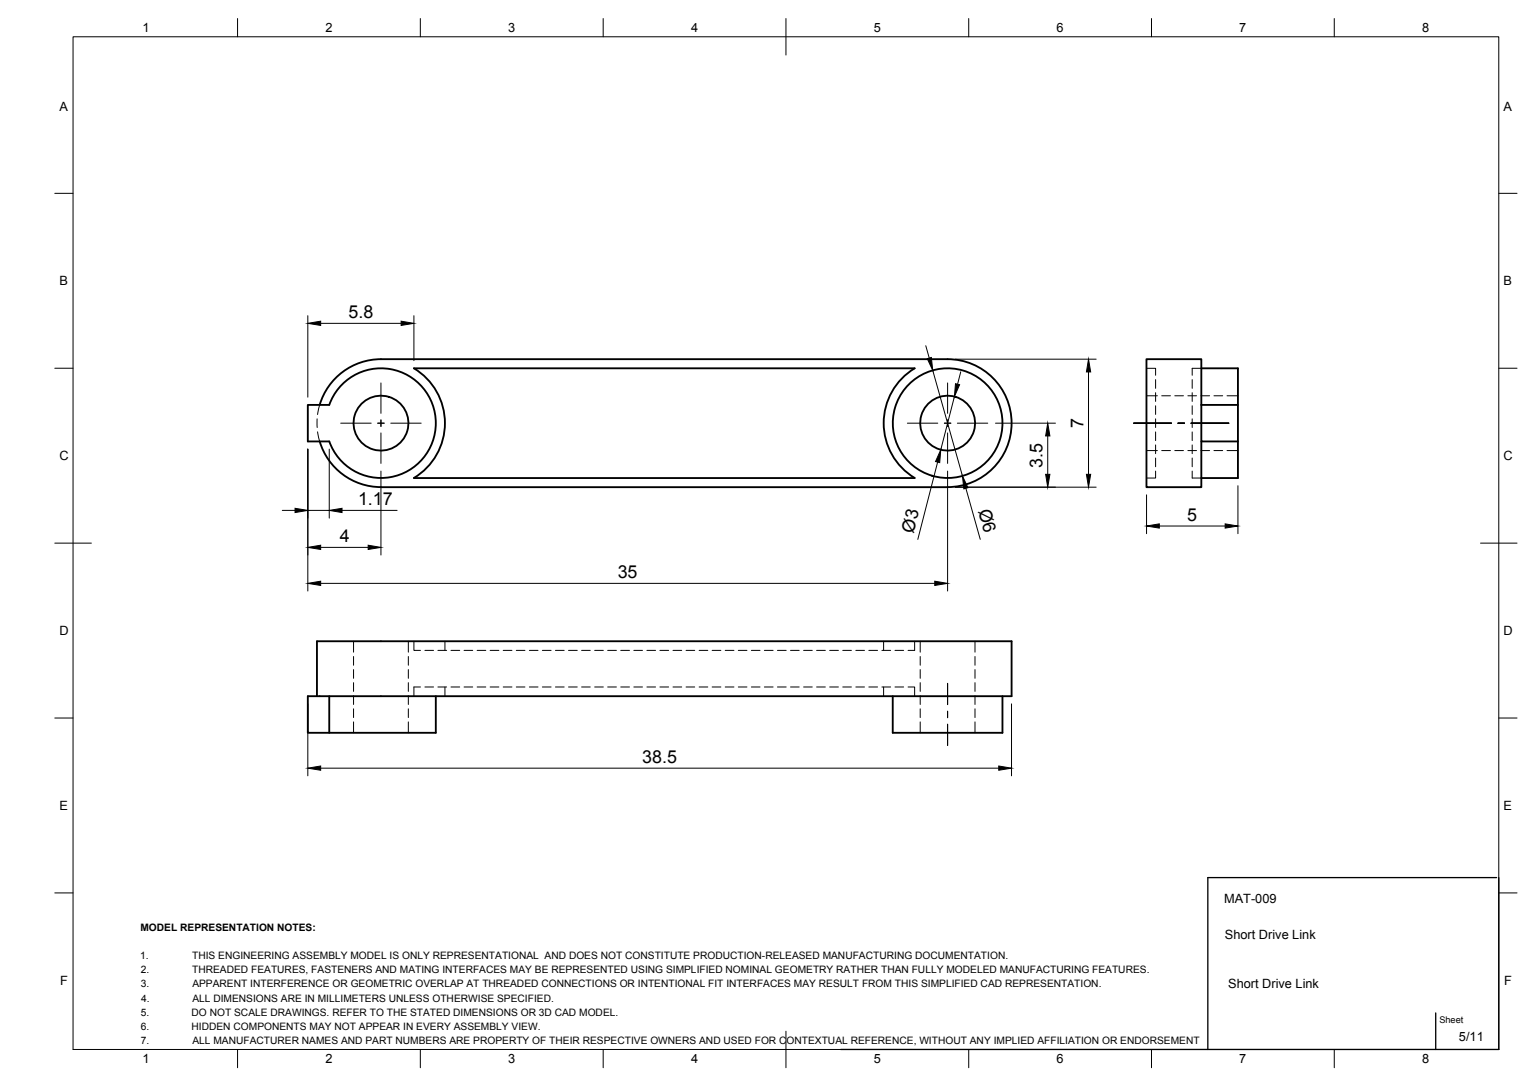
ISO-10303-21;
HEADER;
/* Generated by software containing ST-Developer
 * from STEP Tools, Inc. (www.steptools.com) 
 */

FILE_DESCRIPTION(
/* description */ ('STEP AP214'),
/* implementation_level */ '2;1');

FILE_NAME(
/* name */ 'Short Drive Link.step',
/* time_stamp */ '2026-11-14T05:43:09-08:00',
/* author */ (''),
/* organization */ (''),
/* preprocessor_version */ 'ST-DEVELOPER v20.2',
/* originating_system */ 'Autodesk Translation Framework v15.17.0.0',
/* authorisation */ '');

FILE_SCHEMA (('AUTOMOTIVE_DESIGN { 1 0 10303 214 3 1 1 }'));
ENDSEC;

DATA;
#10=MECHANICAL_DESIGN_GEOMETRIC_PRESENTATION_REPRESENTATION('',(#147),#11933);
#129=SHAPE_REPRESENTATION_RELATIONSHIP('SRR','None',#11989,#138);
#138=ADVANCED_BREP_SHAPE_REPRESENTATION('',(#156),#11925);
#147=STYLED_ITEM('',(#12042),#156);
#156=MANIFOLD_SOLID_BREP('Body1',#6644);
#176=FACE_BOUND('',#714,.T.);
#177=FACE_BOUND('',#715,.T.);
#178=FACE_BOUND('',#717,.T.);
#179=FACE_BOUND('',#718,.T.);
#180=FACE_BOUND('',#719,.T.);
#181=FACE_BOUND('',#737,.T.);
#182=FACE_BOUND('',#739,.T.);
#219=PLANE('',#6821);
#220=PLANE('',#6825);
#221=PLANE('',#6828);
#222=PLANE('',#6830);
#223=PLANE('',#6833);
#224=PLANE('',#6834);
#225=PLANE('',#6835);
#226=PLANE('',#6836);
#227=PLANE('',#6839);
#228=PLANE('',#6840);
#229=PLANE('',#6841);
#230=PLANE('',#6842);
#231=PLANE('',#6845);
#232=PLANE('',#6846);
#233=PLANE('',#6847);
#234=PLANE('',#6848);
#341=FACE_OUTER_BOUND('',#707,.T.);
#342=FACE_OUTER_BOUND('',#708,.T.);
#343=FACE_OUTER_BOUND('',#709,.T.);
#344=FACE_OUTER_BOUND('',#710,.T.);
#345=FACE_OUTER_BOUND('',#711,.T.);
#346=FACE_OUTER_BOUND('',#712,.T.);
#347=FACE_OUTER_BOUND('',#713,.T.);
#348=FACE_OUTER_BOUND('',#716,.T.);
#349=FACE_OUTER_BOUND('',#720,.T.);
#350=FACE_OUTER_BOUND('',#721,.T.);
#351=FACE_OUTER_BOUND('',#722,.T.);
#352=FACE_OUTER_BOUND('',#723,.T.);
#353=FACE_OUTER_BOUND('',#724,.T.);
#354=FACE_OUTER_BOUND('',#725,.T.);
#355=FACE_OUTER_BOUND('',#726,.T.);
#356=FACE_OUTER_BOUND('',#727,.T.);
#357=FACE_OUTER_BOUND('',#728,.T.);
#358=FACE_OUTER_BOUND('',#729,.T.);
#359=FACE_OUTER_BOUND('',#730,.T.);
#360=FACE_OUTER_BOUND('',#731,.T.);
#361=FACE_OUTER_BOUND('',#732,.T.);
#362=FACE_OUTER_BOUND('',#733,.T.);
#363=FACE_OUTER_BOUND('',#734,.T.);
#364=FACE_OUTER_BOUND('',#735,.T.);
#365=FACE_OUTER_BOUND('',#736,.T.);
#366=FACE_OUTER_BOUND('',#738,.T.);
#707=EDGE_LOOP('',(#4232,#4233,#4234,#4235));
#708=EDGE_LOOP('',(#4236,#4237,#4238,#4239));
#709=EDGE_LOOP('',(#4240,#4241,#4242,#4243));
#710=EDGE_LOOP('',(#4244,#4245,#4246,#4247));
#711=EDGE_LOOP('',(#4248,#4249,#4250,#4251));
#712=EDGE_LOOP('',(#4252,#4253,#4254,#4255,#4256,#4257));
#713=EDGE_LOOP('',(#4258,#4259,#4260,#4261,#4262,#4263,#4264,#4265));
#714=EDGE_LOOP('',(#4266,#4267,#4268,#4269));
#715=EDGE_LOOP('',(#4270));
#716=EDGE_LOOP('',(#4271,#4272,#4273,#4274));
#717=EDGE_LOOP('',(#4275));
#718=EDGE_LOOP('',(#4276,#4277,#4278,#4279));
#719=EDGE_LOOP('',(#4280));
#720=EDGE_LOOP('',(#4281,#4282,#4283,#4284));
#721=EDGE_LOOP('',(#4285,#4286,#4287,#4288));
#722=EDGE_LOOP('',(#4289,#4290,#4291,#4292));
#723=EDGE_LOOP('',(#4293,#4294,#4295,#4296));
#724=EDGE_LOOP('',(#4297,#4298,#4299,#4300));
#725=EDGE_LOOP('',(#4301,#4302,#4303,#4304));
#726=EDGE_LOOP('',(#4305,#4306,#4307,#4308));
#727=EDGE_LOOP('',(#4309,#4310,#4311,#4312));
#728=EDGE_LOOP('',(#4313,#4314,#4315,#4316));
#729=EDGE_LOOP('',(#4317,#4318,#4319,#4320));
#730=EDGE_LOOP('',(#4321,#4322,#4323,#4324));
#731=EDGE_LOOP('',(#4325,#4326,#4327,#4328));
#732=EDGE_LOOP('',(#4329,#4330,#4331,#4332,#4333));
#733=EDGE_LOOP('',(#4334,#4335,#4336,#4337));
#734=EDGE_LOOP('',(#4338,#4339,#4340,#4341,#4342));
#735=EDGE_LOOP('',(#4343,#4344,#4345,#4346));
#736=EDGE_LOOP('',(#4347,#4348,#4349,#4350));
#737=EDGE_LOOP('',(#4351));
#738=EDGE_LOOP('',(#4352));
#739=EDGE_LOOP('',(#4353));
#1108=LINE('',#10037,#1570);
#1109=LINE('',#10044,#1571);
#1110=LINE('',#10047,#1572);
#1111=LINE('',#10053,#1573);
#1112=LINE('',#10056,#1574);
#1113=LINE('',#10061,#1575);
#1114=LINE('',#10067,#1576);
#1115=LINE('',#10076,#1577);
#1116=LINE('',#10080,#1578);
#1117=LINE('',#10086,#1579);
#1118=LINE('',#10088,#1580);
#1119=LINE('',#10091,#1581);
#1120=LINE('',#10092,#1582);
#1121=LINE('',#10096,#1583);
#1122=LINE('',#10097,#1584);
#1123=LINE('',#10100,#1585);
#1124=LINE('',#10103,#1586);
#1125=LINE('',#10105,#1587);
#1126=LINE('',#10108,#1588);
#1127=LINE('',#10110,#1589);
#1128=LINE('',#10112,#1590);
#1129=LINE('',#10116,#1591);
#1130=LINE('',#10119,#1592);
#1131=LINE('',#10121,#1593);
#1132=LINE('',#10123,#1594);
#1133=LINE('',#10127,#1595);
#1134=LINE('',#10128,#1596);
#1135=LINE('',#10132,#1597);
#1136=LINE('',#10134,#1598);
#1137=LINE('',#10138,#1599);
#1138=LINE('',#10140,#1600);
#1139=LINE('',#10141,#1601);
#1140=LINE('',#10144,#1602);
#1141=LINE('',#10146,#1603);
#1142=LINE('',#10147,#1604);
#1143=LINE('',#10150,#1605);
#1144=LINE('',#10154,#1606);
#1145=LINE('',#10155,#1607);
#1146=LINE('',#10157,#1608);
#1570=VECTOR('',#7788,3.);
#1571=VECTOR('',#7795,1000.);
#1572=VECTOR('',#7798,1000.);
#1573=VECTOR('',#7803,1000.);
#1574=VECTOR('',#7806,1000.);
#1575=VECTOR('',#7811,1.5);
#1576=VECTOR('',#7818,1.5);
#1577=VECTOR('',#7827,1000.);
#1578=VECTOR('',#7830,1000.);
#1579=VECTOR('',#7837,1000.);
#1580=VECTOR('',#7838,1000.);
#1581=VECTOR('',#7841,1000.);
#1582=VECTOR('',#7842,1000.);
#1583=VECTOR('',#7845,1000.);
#1584=VECTOR('',#7846,1000.);
#1585=VECTOR('',#7849,1000.);
#1586=VECTOR('',#7852,1000.);
#1587=VECTOR('',#7853,1000.);
#1588=VECTOR('',#7856,1000.);
#1589=VECTOR('',#7859,1000.);
#1590=VECTOR('',#7862,1000.);
#1591=VECTOR('',#7867,1000.);
#1592=VECTOR('',#7870,1000.);
#1593=VECTOR('',#7873,1000.);
#1594=VECTOR('',#7876,1000.);
#1595=VECTOR('',#7881,1000.);
#1596=VECTOR('',#7882,1000.);
#1597=VECTOR('',#7887,1000.);
#1598=VECTOR('',#7890,1000.);
#1599=VECTOR('',#7895,1000.);
#1600=VECTOR('',#7896,1000.);
#1601=VECTOR('',#7897,1000.);
#1602=VECTOR('',#7900,1000.);
#1603=VECTOR('',#7901,1000.);
#1604=VECTOR('',#7902,1000.);
#1605=VECTOR('',#7905,1000.);
#1606=VECTOR('',#7910,1000.);
#1607=VECTOR('',#7911,1000.);
#1608=VECTOR('',#7914,1000.);
#2020=CIRCLE('',#6802,3.);
#2021=CIRCLE('',#6803,3.);
#2022=CIRCLE('',#6805,3.5);
#2023=CIRCLE('',#6806,3.5);
#2024=CIRCLE('',#6808,3.5);
#2025=CIRCLE('',#6809,3.5);
#2026=CIRCLE('',#6811,1.5);
#2027=CIRCLE('',#6812,1.5);
#2028=CIRCLE('',#6814,1.5);
#2029=CIRCLE('',#6815,1.5);
#2030=CIRCLE('',#6817,3.5);
#2031=CIRCLE('',#6818,3.5);
#2032=CIRCLE('',#6819,3.5);
#2033=CIRCLE('',#6820,3.5);
#2034=CIRCLE('',#6822,3.);
#2035=CIRCLE('',#6823,3.5);
#2036=CIRCLE('',#6824,3.5);
#2037=CIRCLE('',#6826,3.5);
#2038=CIRCLE('',#6827,3.5);
#2039=CIRCLE('',#6832,3.5);
#2040=CIRCLE('',#6838,3.5);
#2041=CIRCLE('',#6844,3.);
#2541=VERTEX_POINT('',#10034);
#2542=VERTEX_POINT('',#10036);
#2543=VERTEX_POINT('',#10040);
#2544=VERTEX_POINT('',#10041);
#2545=VERTEX_POINT('',#10043);
#2546=VERTEX_POINT('',#10045);
#2547=VERTEX_POINT('',#10049);
#2548=VERTEX_POINT('',#10050);
#2549=VERTEX_POINT('',#10052);
#2550=VERTEX_POINT('',#10054);
#2551=VERTEX_POINT('',#10058);
#2552=VERTEX_POINT('',#10060);
#2553=VERTEX_POINT('',#10064);
#2554=VERTEX_POINT('',#10066);
#2555=VERTEX_POINT('',#10070);
#2556=VERTEX_POINT('',#10071);
#2557=VERTEX_POINT('',#10073);
#2558=VERTEX_POINT('',#10075);
#2559=VERTEX_POINT('',#10077);
#2560=VERTEX_POINT('',#10079);
#2561=VERTEX_POINT('',#10083);
#2562=VERTEX_POINT('',#10084);
#2563=VERTEX_POINT('',#10087);
#2564=VERTEX_POINT('',#10089);
#2565=VERTEX_POINT('',#10093);
#2566=VERTEX_POINT('',#10094);
#2567=VERTEX_POINT('',#10099);
#2568=VERTEX_POINT('',#10101);
#2569=VERTEX_POINT('',#10104);
#2570=VERTEX_POINT('',#10106);
#2571=VERTEX_POINT('',#10115);
#2572=VERTEX_POINT('',#10117);
#2573=VERTEX_POINT('',#10126);
#2574=VERTEX_POINT('',#10130);
#2575=VERTEX_POINT('',#10137);
#2576=VERTEX_POINT('',#10139);
#2577=VERTEX_POINT('',#10143);
#2578=VERTEX_POINT('',#10145);
#2579=VERTEX_POINT('',#10149);
#2580=VERTEX_POINT('',#10153);
#3205=EDGE_CURVE('',#2541,#2541,#2020,.T.);
#3206=EDGE_CURVE('',#2541,#2542,#1108,.T.);
#3207=EDGE_CURVE('',#2542,#2542,#2021,.T.);
#3208=EDGE_CURVE('',#2543,#2544,#2022,.T.);
#3209=EDGE_CURVE('',#2544,#2545,#1109,.T.);
#3210=EDGE_CURVE('',#2546,#2545,#2023,.T.);
#3211=EDGE_CURVE('',#2543,#2546,#1110,.T.);
#3212=EDGE_CURVE('',#2547,#2548,#2024,.T.);
#3213=EDGE_CURVE('',#2547,#2549,#1111,.T.);
#3214=EDGE_CURVE('',#2549,#2550,#2025,.T.);
#3215=EDGE_CURVE('',#2548,#2550,#1112,.T.);
#3216=EDGE_CURVE('',#2551,#2551,#2026,.T.);
#3217=EDGE_CURVE('',#2551,#2552,#1113,.T.);
#3218=EDGE_CURVE('',#2552,#2552,#2027,.T.);
#3219=EDGE_CURVE('',#2553,#2553,#2028,.T.);
#3220=EDGE_CURVE('',#2553,#2554,#1114,.T.);
#3221=EDGE_CURVE('',#2554,#2554,#2029,.T.);
#3222=EDGE_CURVE('',#2555,#2556,#2030,.T.);
#3223=EDGE_CURVE('',#2557,#2555,#2031,.T.);
#3224=EDGE_CURVE('',#2557,#2558,#1115,.T.);
#3225=EDGE_CURVE('',#2558,#2559,#2032,.T.);
#3226=EDGE_CURVE('',#2560,#2559,#1116,.T.);
#3227=EDGE_CURVE('',#2556,#2560,#2033,.T.);
#3228=EDGE_CURVE('',#2561,#2562,#2034,.T.);
#3229=EDGE_CURVE('',#2561,#2556,#1117,.T.);
#3230=EDGE_CURVE('',#2560,#2563,#1118,.T.);
#3231=EDGE_CURVE('',#2563,#2564,#2035,.T.);
#3232=EDGE_CURVE('',#2564,#2557,#1119,.T.);
#3233=EDGE_CURVE('',#2562,#2555,#1120,.T.);
#3234=EDGE_CURVE('',#2565,#2566,#2036,.T.);
#3235=EDGE_CURVE('',#2550,#2565,#1121,.T.);
#3236=EDGE_CURVE('',#2566,#2549,#1122,.T.);
#3237=EDGE_CURVE('',#2567,#2558,#1123,.T.);
#3238=EDGE_CURVE('',#2568,#2567,#2037,.T.);
#3239=EDGE_CURVE('',#2559,#2568,#1124,.T.);
#3240=EDGE_CURVE('',#2545,#2569,#1125,.T.);
#3241=EDGE_CURVE('',#2569,#2570,#2038,.T.);
#3242=EDGE_CURVE('',#2570,#2546,#1126,.T.);
#3243=EDGE_CURVE('',#2563,#2568,#1127,.T.);
#3244=EDGE_CURVE('',#2564,#2567,#1128,.T.);
#3245=EDGE_CURVE('',#2571,#2566,#1129,.T.);
#3246=EDGE_CURVE('',#2572,#2571,#2039,.T.);
#3247=EDGE_CURVE('',#2572,#2565,#1130,.T.);
#3248=EDGE_CURVE('',#2548,#2572,#1131,.T.);
#3249=EDGE_CURVE('',#2571,#2547,#1132,.T.);
#3250=EDGE_CURVE('',#2544,#2573,#1133,.T.);
#3251=EDGE_CURVE('',#2573,#2569,#1134,.T.);
#3252=EDGE_CURVE('',#2573,#2574,#2040,.T.);
#3253=EDGE_CURVE('',#2574,#2570,#1135,.T.);
#3254=EDGE_CURVE('',#2574,#2543,#1136,.T.);
#3255=EDGE_CURVE('',#2555,#2575,#1137,.T.);
#3256=EDGE_CURVE('',#2556,#2576,#1138,.T.);
#3257=EDGE_CURVE('',#2575,#2576,#1139,.T.);
#3258=EDGE_CURVE('',#2577,#2561,#1140,.T.);
#3259=EDGE_CURVE('',#2577,#2578,#1141,.T.);
#3260=EDGE_CURVE('',#2578,#2576,#1142,.T.);
#3261=EDGE_CURVE('',#2579,#2562,#1143,.T.);
#3262=EDGE_CURVE('',#2577,#2579,#2041,.T.);
#3263=EDGE_CURVE('',#2580,#2575,#1144,.T.);
#3264=EDGE_CURVE('',#2579,#2580,#1145,.T.);
#3265=EDGE_CURVE('',#2580,#2578,#1146,.T.);
#4232=ORIENTED_EDGE('',*,*,#3205,.T.);
#4233=ORIENTED_EDGE('',*,*,#3206,.T.);
#4234=ORIENTED_EDGE('',*,*,#3207,.F.);
#4235=ORIENTED_EDGE('',*,*,#3206,.F.);
#4236=ORIENTED_EDGE('',*,*,#3208,.T.);
#4237=ORIENTED_EDGE('',*,*,#3209,.T.);
#4238=ORIENTED_EDGE('',*,*,#3210,.F.);
#4239=ORIENTED_EDGE('',*,*,#3211,.F.);
#4240=ORIENTED_EDGE('',*,*,#3212,.F.);
#4241=ORIENTED_EDGE('',*,*,#3213,.T.);
#4242=ORIENTED_EDGE('',*,*,#3214,.T.);
#4243=ORIENTED_EDGE('',*,*,#3215,.F.);
#4244=ORIENTED_EDGE('',*,*,#3216,.F.);
#4245=ORIENTED_EDGE('',*,*,#3217,.T.);
#4246=ORIENTED_EDGE('',*,*,#3218,.F.);
#4247=ORIENTED_EDGE('',*,*,#3217,.F.);
#4248=ORIENTED_EDGE('',*,*,#3219,.F.);
#4249=ORIENTED_EDGE('',*,*,#3220,.T.);
#4250=ORIENTED_EDGE('',*,*,#3221,.F.);
#4251=ORIENTED_EDGE('',*,*,#3220,.F.);
#4252=ORIENTED_EDGE('',*,*,#3222,.F.);
#4253=ORIENTED_EDGE('',*,*,#3223,.F.);
#4254=ORIENTED_EDGE('',*,*,#3224,.T.);
#4255=ORIENTED_EDGE('',*,*,#3225,.T.);
#4256=ORIENTED_EDGE('',*,*,#3226,.F.);
#4257=ORIENTED_EDGE('',*,*,#3227,.F.);
#4258=ORIENTED_EDGE('',*,*,#3228,.F.);
#4259=ORIENTED_EDGE('',*,*,#3229,.T.);
#4260=ORIENTED_EDGE('',*,*,#3227,.T.);
#4261=ORIENTED_EDGE('',*,*,#3230,.T.);
#4262=ORIENTED_EDGE('',*,*,#3231,.T.);
#4263=ORIENTED_EDGE('',*,*,#3232,.T.);
#4264=ORIENTED_EDGE('',*,*,#3223,.T.);
#4265=ORIENTED_EDGE('',*,*,#3233,.F.);
#4266=ORIENTED_EDGE('',*,*,#3234,.F.);
#4267=ORIENTED_EDGE('',*,*,#3235,.F.);
#4268=ORIENTED_EDGE('',*,*,#3214,.F.);
#4269=ORIENTED_EDGE('',*,*,#3236,.F.);
#4270=ORIENTED_EDGE('',*,*,#3205,.F.);
#4271=ORIENTED_EDGE('',*,*,#3225,.F.);
#4272=ORIENTED_EDGE('',*,*,#3237,.F.);
#4273=ORIENTED_EDGE('',*,*,#3238,.F.);
#4274=ORIENTED_EDGE('',*,*,#3239,.F.);
#4275=ORIENTED_EDGE('',*,*,#3221,.T.);
#4276=ORIENTED_EDGE('',*,*,#3210,.T.);
#4277=ORIENTED_EDGE('',*,*,#3240,.T.);
#4278=ORIENTED_EDGE('',*,*,#3241,.T.);
#4279=ORIENTED_EDGE('',*,*,#3242,.T.);
#4280=ORIENTED_EDGE('',*,*,#3218,.T.);
#4281=ORIENTED_EDGE('',*,*,#3239,.T.);
#4282=ORIENTED_EDGE('',*,*,#3243,.F.);
#4283=ORIENTED_EDGE('',*,*,#3230,.F.);
#4284=ORIENTED_EDGE('',*,*,#3226,.T.);
#4285=ORIENTED_EDGE('',*,*,#3238,.T.);
#4286=ORIENTED_EDGE('',*,*,#3244,.F.);
#4287=ORIENTED_EDGE('',*,*,#3231,.F.);
#4288=ORIENTED_EDGE('',*,*,#3243,.T.);
#4289=ORIENTED_EDGE('',*,*,#3237,.T.);
#4290=ORIENTED_EDGE('',*,*,#3224,.F.);
#4291=ORIENTED_EDGE('',*,*,#3232,.F.);
#4292=ORIENTED_EDGE('',*,*,#3244,.T.);
#4293=ORIENTED_EDGE('',*,*,#3234,.T.);
#4294=ORIENTED_EDGE('',*,*,#3245,.F.);
#4295=ORIENTED_EDGE('',*,*,#3246,.F.);
#4296=ORIENTED_EDGE('',*,*,#3247,.T.);
#4297=ORIENTED_EDGE('',*,*,#3235,.T.);
#4298=ORIENTED_EDGE('',*,*,#3247,.F.);
#4299=ORIENTED_EDGE('',*,*,#3248,.F.);
#4300=ORIENTED_EDGE('',*,*,#3215,.T.);
#4301=ORIENTED_EDGE('',*,*,#3236,.T.);
#4302=ORIENTED_EDGE('',*,*,#3213,.F.);
#4303=ORIENTED_EDGE('',*,*,#3249,.F.);
#4304=ORIENTED_EDGE('',*,*,#3245,.T.);
#4305=ORIENTED_EDGE('',*,*,#3246,.T.);
#4306=ORIENTED_EDGE('',*,*,#3249,.T.);
#4307=ORIENTED_EDGE('',*,*,#3212,.T.);
#4308=ORIENTED_EDGE('',*,*,#3248,.T.);
#4309=ORIENTED_EDGE('',*,*,#3240,.F.);
#4310=ORIENTED_EDGE('',*,*,#3209,.F.);
#4311=ORIENTED_EDGE('',*,*,#3250,.T.);
#4312=ORIENTED_EDGE('',*,*,#3251,.T.);
#4313=ORIENTED_EDGE('',*,*,#3241,.F.);
#4314=ORIENTED_EDGE('',*,*,#3251,.F.);
#4315=ORIENTED_EDGE('',*,*,#3252,.T.);
#4316=ORIENTED_EDGE('',*,*,#3253,.T.);
#4317=ORIENTED_EDGE('',*,*,#3242,.F.);
#4318=ORIENTED_EDGE('',*,*,#3253,.F.);
#4319=ORIENTED_EDGE('',*,*,#3254,.T.);
#4320=ORIENTED_EDGE('',*,*,#3211,.T.);
#4321=ORIENTED_EDGE('',*,*,#3208,.F.);
#4322=ORIENTED_EDGE('',*,*,#3254,.F.);
#4323=ORIENTED_EDGE('',*,*,#3252,.F.);
#4324=ORIENTED_EDGE('',*,*,#3250,.F.);
#4325=ORIENTED_EDGE('',*,*,#3255,.F.);
#4326=ORIENTED_EDGE('',*,*,#3222,.T.);
#4327=ORIENTED_EDGE('',*,*,#3256,.T.);
#4328=ORIENTED_EDGE('',*,*,#3257,.F.);
#4329=ORIENTED_EDGE('',*,*,#3229,.F.);
#4330=ORIENTED_EDGE('',*,*,#3258,.F.);
#4331=ORIENTED_EDGE('',*,*,#3259,.T.);
#4332=ORIENTED_EDGE('',*,*,#3260,.T.);
#4333=ORIENTED_EDGE('',*,*,#3256,.F.);
#4334=ORIENTED_EDGE('',*,*,#3228,.T.);
#4335=ORIENTED_EDGE('',*,*,#3261,.F.);
#4336=ORIENTED_EDGE('',*,*,#3262,.F.);
#4337=ORIENTED_EDGE('',*,*,#3258,.T.);
#4338=ORIENTED_EDGE('',*,*,#3233,.T.);
#4339=ORIENTED_EDGE('',*,*,#3255,.T.);
#4340=ORIENTED_EDGE('',*,*,#3263,.F.);
#4341=ORIENTED_EDGE('',*,*,#3264,.F.);
#4342=ORIENTED_EDGE('',*,*,#3261,.T.);
#4343=ORIENTED_EDGE('',*,*,#3257,.T.);
#4344=ORIENTED_EDGE('',*,*,#3260,.F.);
#4345=ORIENTED_EDGE('',*,*,#3265,.F.);
#4346=ORIENTED_EDGE('',*,*,#3263,.T.);
#4347=ORIENTED_EDGE('',*,*,#3259,.F.);
#4348=ORIENTED_EDGE('',*,*,#3262,.T.);
#4349=ORIENTED_EDGE('',*,*,#3264,.T.);
#4350=ORIENTED_EDGE('',*,*,#3265,.T.);
#4351=ORIENTED_EDGE('',*,*,#3219,.T.);
#4352=ORIENTED_EDGE('',*,*,#3207,.T.);
#4353=ORIENTED_EDGE('',*,*,#3216,.T.);
#6058=CYLINDRICAL_SURFACE('',#6801,3.);
#6059=CYLINDRICAL_SURFACE('',#6804,3.5);
#6060=CYLINDRICAL_SURFACE('',#6807,3.5);
#6061=CYLINDRICAL_SURFACE('',#6810,1.5);
#6062=CYLINDRICAL_SURFACE('',#6813,1.5);
#6063=CYLINDRICAL_SURFACE('',#6816,3.5);
#6064=CYLINDRICAL_SURFACE('',#6829,3.5);
#6065=CYLINDRICAL_SURFACE('',#6831,3.5);
#6066=CYLINDRICAL_SURFACE('',#6837,3.5);
#6067=CYLINDRICAL_SURFACE('',#6843,3.);
#6311=ADVANCED_FACE('',(#341),#6058,.T.);
#6312=ADVANCED_FACE('',(#342),#6059,.T.);
#6313=ADVANCED_FACE('',(#343),#6060,.T.);
#6314=ADVANCED_FACE('',(#344),#6061,.F.);
#6315=ADVANCED_FACE('',(#345),#6062,.F.);
#6316=ADVANCED_FACE('',(#346),#6063,.T.);
#6317=ADVANCED_FACE('',(#347,#176,#177),#219,.T.);
#6318=ADVANCED_FACE('',(#348,#178,#179,#180),#220,.F.);
#6319=ADVANCED_FACE('',(#349),#221,.F.);
#6320=ADVANCED_FACE('',(#350),#6064,.T.);
#6321=ADVANCED_FACE('',(#351),#222,.F.);
#6322=ADVANCED_FACE('',(#352),#6065,.T.);
#6323=ADVANCED_FACE('',(#353),#223,.F.);
#6324=ADVANCED_FACE('',(#354),#224,.F.);
#6325=ADVANCED_FACE('',(#355),#225,.T.);
#6326=ADVANCED_FACE('',(#356),#226,.T.);
#6327=ADVANCED_FACE('',(#357),#6066,.T.);
#6328=ADVANCED_FACE('',(#358),#227,.T.);
#6329=ADVANCED_FACE('',(#359),#228,.T.);
#6330=ADVANCED_FACE('',(#360),#229,.F.);
#6331=ADVANCED_FACE('',(#361),#230,.T.);
#6332=ADVANCED_FACE('',(#362),#6067,.T.);
#6333=ADVANCED_FACE('',(#363),#231,.F.);
#6334=ADVANCED_FACE('',(#364),#232,.F.);
#6335=ADVANCED_FACE('',(#365,#181),#233,.T.);
#6336=ADVANCED_FACE('',(#366,#182),#234,.T.);
#6644=CLOSED_SHELL('',(#6311,#6312,#6313,#6314,#6315,#6316,#6317,#6318,
#6319,#6320,#6321,#6322,#6323,#6324,#6325,#6326,#6327,#6328,#6329,#6330,
#6331,#6332,#6333,#6334,#6335,#6336));
#6800=AXIS2_PLACEMENT_3D('',#10032,#7782,#7783);
#6801=AXIS2_PLACEMENT_3D('',#10033,#7784,#7785);
#6802=AXIS2_PLACEMENT_3D('',#10035,#7786,#7787);
#6803=AXIS2_PLACEMENT_3D('',#10038,#7789,#7790);
#6804=AXIS2_PLACEMENT_3D('',#10039,#7791,#7792);
#6805=AXIS2_PLACEMENT_3D('',#10042,#7793,#7794);
#6806=AXIS2_PLACEMENT_3D('',#10046,#7796,#7797);
#6807=AXIS2_PLACEMENT_3D('',#10048,#7799,#7800);
#6808=AXIS2_PLACEMENT_3D('',#10051,#7801,#7802);
#6809=AXIS2_PLACEMENT_3D('',#10055,#7804,#7805);
#6810=AXIS2_PLACEMENT_3D('',#10057,#7807,#7808);
#6811=AXIS2_PLACEMENT_3D('',#10059,#7809,#7810);
#6812=AXIS2_PLACEMENT_3D('',#10062,#7812,#7813);
#6813=AXIS2_PLACEMENT_3D('',#10063,#7814,#7815);
#6814=AXIS2_PLACEMENT_3D('',#10065,#7816,#7817);
#6815=AXIS2_PLACEMENT_3D('',#10068,#7819,#7820);
#6816=AXIS2_PLACEMENT_3D('',#10069,#7821,#7822);
#6817=AXIS2_PLACEMENT_3D('',#10072,#7823,#7824);
#6818=AXIS2_PLACEMENT_3D('',#10074,#7825,#7826);
#6819=AXIS2_PLACEMENT_3D('',#10078,#7828,#7829);
#6820=AXIS2_PLACEMENT_3D('',#10081,#7831,#7832);
#6821=AXIS2_PLACEMENT_3D('',#10082,#7833,#7834);
#6822=AXIS2_PLACEMENT_3D('',#10085,#7835,#7836);
#6823=AXIS2_PLACEMENT_3D('',#10090,#7839,#7840);
#6824=AXIS2_PLACEMENT_3D('',#10095,#7843,#7844);
#6825=AXIS2_PLACEMENT_3D('',#10098,#7847,#7848);
#6826=AXIS2_PLACEMENT_3D('',#10102,#7850,#7851);
#6827=AXIS2_PLACEMENT_3D('',#10107,#7854,#7855);
#6828=AXIS2_PLACEMENT_3D('',#10109,#7857,#7858);
#6829=AXIS2_PLACEMENT_3D('',#10111,#7860,#7861);
#6830=AXIS2_PLACEMENT_3D('',#10113,#7863,#7864);
#6831=AXIS2_PLACEMENT_3D('',#10114,#7865,#7866);
#6832=AXIS2_PLACEMENT_3D('',#10118,#7868,#7869);
#6833=AXIS2_PLACEMENT_3D('',#10120,#7871,#7872);
#6834=AXIS2_PLACEMENT_3D('',#10122,#7874,#7875);
#6835=AXIS2_PLACEMENT_3D('',#10124,#7877,#7878);
#6836=AXIS2_PLACEMENT_3D('',#10125,#7879,#7880);
#6837=AXIS2_PLACEMENT_3D('',#10129,#7883,#7884);
#6838=AXIS2_PLACEMENT_3D('',#10131,#7885,#7886);
#6839=AXIS2_PLACEMENT_3D('',#10133,#7888,#7889);
#6840=AXIS2_PLACEMENT_3D('',#10135,#7891,#7892);
#6841=AXIS2_PLACEMENT_3D('',#10136,#7893,#7894);
#6842=AXIS2_PLACEMENT_3D('',#10142,#7898,#7899);
#6843=AXIS2_PLACEMENT_3D('',#10148,#7903,#7904);
#6844=AXIS2_PLACEMENT_3D('',#10151,#7906,#7907);
#6845=AXIS2_PLACEMENT_3D('',#10152,#7908,#7909);
#6846=AXIS2_PLACEMENT_3D('',#10156,#7912,#7913);
#6847=AXIS2_PLACEMENT_3D('',#10158,#7915,#7916);
#6848=AXIS2_PLACEMENT_3D('',#10159,#7917,#7918);
#7782=DIRECTION('axis',(0.,0.,1.));
#7783=DIRECTION('refdir',(1.,0.,0.));
#7784=DIRECTION('center_axis',(0.,0.,-1.));
#7785=DIRECTION('ref_axis',(-1.,0.,0.));
#7786=DIRECTION('center_axis',(0.,0.,1.));
#7787=DIRECTION('ref_axis',(1.,0.,0.));
#7788=DIRECTION('',(0.,0.,1.));
#7789=DIRECTION('center_axis',(0.,0.,1.));
#7790=DIRECTION('ref_axis',(1.,0.,0.));
#7791=DIRECTION('center_axis',(0.,0.,-1.));
#7792=DIRECTION('ref_axis',(-1.,0.,0.));
#7793=DIRECTION('center_axis',(0.,0.,-1.));
#7794=DIRECTION('ref_axis',(1.,0.,0.));
#7795=DIRECTION('',(0.,0.,-1.));
#7796=DIRECTION('center_axis',(0.,0.,-1.));
#7797=DIRECTION('ref_axis',(1.,0.,0.));
#7798=DIRECTION('',(0.,0.,-1.));
#7799=DIRECTION('center_axis',(0.,0.,1.));
#7800=DIRECTION('ref_axis',(1.,0.,0.));
#7801=DIRECTION('center_axis',(0.,0.,-1.));
#7802=DIRECTION('ref_axis',(1.,0.,0.));
#7803=DIRECTION('',(0.,0.,1.));
#7804=DIRECTION('center_axis',(0.,0.,-1.));
#7805=DIRECTION('ref_axis',(1.,0.,0.));
#7806=DIRECTION('',(0.,0.,1.));
#7807=DIRECTION('center_axis',(0.,0.,-1.));
#7808=DIRECTION('ref_axis',(-1.,0.,0.));
#7809=DIRECTION('center_axis',(0.,0.,-1.));
#7810=DIRECTION('ref_axis',(1.,0.,0.));
#7811=DIRECTION('',(0.,0.,-1.));
#7812=DIRECTION('center_axis',(0.,0.,1.));
#7813=DIRECTION('ref_axis',(1.,0.,0.));
#7814=DIRECTION('center_axis',(0.,0.,-1.));
#7815=DIRECTION('ref_axis',(-1.,0.,0.));
#7816=DIRECTION('center_axis',(0.,0.,-1.));
#7817=DIRECTION('ref_axis',(1.,0.,0.));
#7818=DIRECTION('',(0.,0.,-1.));
#7819=DIRECTION('center_axis',(0.,0.,1.));
#7820=DIRECTION('ref_axis',(1.,0.,0.));
#7821=DIRECTION('center_axis',(0.,0.,-1.));
#7822=DIRECTION('ref_axis',(-1.,0.,0.));
#7823=DIRECTION('center_axis',(0.,0.,1.));
#7824=DIRECTION('ref_axis',(1.,0.,0.));
#7825=DIRECTION('center_axis',(0.,0.,1.));
#7826=DIRECTION('ref_axis',(1.,0.,0.));
#7827=DIRECTION('',(0.,0.,-1.));
#7828=DIRECTION('center_axis',(0.,0.,1.));
#7829=DIRECTION('ref_axis',(1.,0.,0.));
#7830=DIRECTION('',(0.,0.,-1.));
#7831=DIRECTION('center_axis',(0.,0.,1.));
#7832=DIRECTION('ref_axis',(1.,0.,0.));
#7833=DIRECTION('center_axis',(0.,0.,1.));
#7834=DIRECTION('ref_axis',(1.,0.,0.));
#7835=DIRECTION('center_axis',(0.,0.,1.));
#7836=DIRECTION('ref_axis',(1.,0.,0.));
#7837=DIRECTION('',(-1.,0.,0.));
#7838=DIRECTION('',(1.,-1.39897054514259E-17,0.));
#7839=DIRECTION('center_axis',(0.,0.,1.));
#7840=DIRECTION('ref_axis',(1.,0.,0.));
#7841=DIRECTION('',(-1.,0.,0.));
#7842=DIRECTION('',(-1.,0.,0.));
#7843=DIRECTION('center_axis',(0.,0.,-1.));
#7844=DIRECTION('ref_axis',(1.,0.,0.));
#7845=DIRECTION('',(1.,3.16619526353726E-17,0.));
#7846=DIRECTION('',(-1.,3.16619526353726E-17,0.));
#7847=DIRECTION('center_axis',(0.,0.,1.));
#7848=DIRECTION('ref_axis',(1.,0.,0.));
#7849=DIRECTION('',(-1.,0.,0.));
#7850=DIRECTION('center_axis',(0.,0.,1.));
#7851=DIRECTION('ref_axis',(1.,0.,0.));
#7852=DIRECTION('',(1.,-1.39897054514259E-17,0.));
#7853=DIRECTION('',(-1.,3.16619526353726E-17,0.));
#7854=DIRECTION('center_axis',(0.,0.,-1.));
#7855=DIRECTION('ref_axis',(1.,0.,0.));
#7856=DIRECTION('',(1.,3.16619526353726E-17,0.));
#7857=DIRECTION('center_axis',(1.39897054514259E-17,1.,0.));
#7858=DIRECTION('ref_axis',(-1.,1.39897054514259E-17,0.));
#7859=DIRECTION('',(0.,0.,-1.));
#7860=DIRECTION('center_axis',(0.,0.,-1.));
#7861=DIRECTION('ref_axis',(1.,1.22464679914735E-16,0.));
#7862=DIRECTION('',(0.,0.,-1.));
#7863=DIRECTION('center_axis',(0.,-1.,0.));
#7864=DIRECTION('ref_axis',(0.,0.,-1.));
#7865=DIRECTION('center_axis',(0.,0.,1.));
#7866=DIRECTION('ref_axis',(-1.,1.22464679914735E-16,0.));
#7867=DIRECTION('',(0.,0.,1.));
#7868=DIRECTION('center_axis',(0.,0.,-1.));
#7869=DIRECTION('ref_axis',(1.,0.,0.));
#7870=DIRECTION('',(0.,0.,1.));
#7871=DIRECTION('center_axis',(3.16619526353726E-17,-1.,0.));
#7872=DIRECTION('ref_axis',(1.,3.16619526353726E-17,0.));
#7873=DIRECTION('',(1.,3.16619526353726E-17,0.));
#7874=DIRECTION('center_axis',(3.16619526353726E-17,1.,0.));
#7875=DIRECTION('ref_axis',(-1.,3.16619526353726E-17,0.));
#7876=DIRECTION('',(-1.,3.16619526353726E-17,0.));
#7877=DIRECTION('center_axis',(0.,0.,1.));
#7878=DIRECTION('ref_axis',(1.,0.,0.));
#7879=DIRECTION('center_axis',(-3.16619526353726E-17,-1.,0.));
#7880=DIRECTION('ref_axis',(1.,-3.16619526353726E-17,0.));
#7881=DIRECTION('',(-1.,3.16619526353726E-17,0.));
#7882=DIRECTION('',(0.,0.,-1.));
#7883=DIRECTION('center_axis',(0.,0.,-1.));
#7884=DIRECTION('ref_axis',(1.,1.22464679914735E-16,0.));
#7885=DIRECTION('center_axis',(0.,0.,-1.));
#7886=DIRECTION('ref_axis',(1.,0.,0.));
#7887=DIRECTION('',(0.,0.,-1.));
#7888=DIRECTION('center_axis',(-3.16619526353726E-17,1.,0.));
#7889=DIRECTION('ref_axis',(-1.,-3.16619526353726E-17,0.));
#7890=DIRECTION('',(1.,3.16619526353726E-17,0.));
#7891=DIRECTION('center_axis',(0.,0.,-1.));
#7892=DIRECTION('ref_axis',(1.,0.,0.));
#7893=DIRECTION('center_axis',(0.,0.,1.));
#7894=DIRECTION('ref_axis',(1.,0.,0.));
#7895=DIRECTION('',(-1.,0.,0.));
#7896=DIRECTION('',(-1.,0.,0.));
#7897=DIRECTION('',(0.,-1.,0.));
#7898=DIRECTION('center_axis',(0.,-1.,0.));
#7899=DIRECTION('ref_axis',(0.,0.,-1.));
#7900=DIRECTION('',(0.,0.,-1.));
#7901=DIRECTION('',(-1.,0.,0.));
#7902=DIRECTION('',(0.,0.,-1.));
#7903=DIRECTION('center_axis',(0.,0.,-1.));
#7904=DIRECTION('ref_axis',(1.,1.22464679914735E-16,0.));
#7905=DIRECTION('',(0.,0.,-1.));
#7906=DIRECTION('center_axis',(0.,0.,1.));
#7907=DIRECTION('ref_axis',(1.,0.,0.));
#7908=DIRECTION('center_axis',(0.,-1.,0.));
#7909=DIRECTION('ref_axis',(0.,0.,-1.));
#7910=DIRECTION('',(0.,0.,-1.));
#7911=DIRECTION('',(-1.,0.,0.));
#7912=DIRECTION('center_axis',(1.,0.,0.));
#7913=DIRECTION('ref_axis',(0.,0.,-1.));
#7914=DIRECTION('',(0.,-1.,0.));
#7915=DIRECTION('center_axis',(0.,0.,1.));
#7916=DIRECTION('ref_axis',(1.,0.,0.));
#7917=DIRECTION('center_axis',(0.,0.,1.));
#7918=DIRECTION('ref_axis',(1.,0.,0.));
#10032=CARTESIAN_POINT('',(0.,0.,0.));
#10033=CARTESIAN_POINT('Origin',(31.,0.,5.));
#10034=CARTESIAN_POINT('',(34.,-3.67394039744206E-16,3.));
#10035=CARTESIAN_POINT('Origin',(31.,0.,3.));
#10036=CARTESIAN_POINT('',(34.,-3.67394039744206E-16,5.));
#10037=CARTESIAN_POINT('',(34.,-3.67394039744206E-16,5.));
#10038=CARTESIAN_POINT('Origin',(31.,0.,5.));
#10039=CARTESIAN_POINT('Origin',(31.,0.,0.5));
#10040=CARTESIAN_POINT('',(29.197224362268,-3.,0.5));
#10041=CARTESIAN_POINT('',(29.197224362268,3.,0.5));
#10042=CARTESIAN_POINT('Origin',(31.,0.,0.5));
#10043=CARTESIAN_POINT('',(29.197224362268,3.,0.));
#10044=CARTESIAN_POINT('',(29.197224362268,3.,0.5));
#10045=CARTESIAN_POINT('',(29.197224362268,-3.,0.));
#10046=CARTESIAN_POINT('Origin',(31.,0.,0.));
#10047=CARTESIAN_POINT('',(29.197224362268,-3.,0.5));
#10048=CARTESIAN_POINT('Origin',(0.,0.,2.5));
#10049=CARTESIAN_POINT('',(1.80277563773199,3.,2.5));
#10050=CARTESIAN_POINT('',(1.802775637732,-3.,2.5));
#10051=CARTESIAN_POINT('Origin',(0.,0.,2.5));
#10052=CARTESIAN_POINT('',(1.80277563773199,3.,3.));
#10053=CARTESIAN_POINT('',(1.80277563773199,3.,2.5));
#10054=CARTESIAN_POINT('',(1.802775637732,-3.,3.));
#10055=CARTESIAN_POINT('Origin',(0.,0.,3.));
#10056=CARTESIAN_POINT('',(1.802775637732,-3.,2.5));
#10057=CARTESIAN_POINT('Origin',(31.,0.,3.));
#10058=CARTESIAN_POINT('',(32.5,-1.83697019872104E-16,5.));
#10059=CARTESIAN_POINT('Origin',(31.,0.,5.));
#10060=CARTESIAN_POINT('',(32.5,-1.83697019872104E-16,0.));
#10061=CARTESIAN_POINT('',(32.5,-1.83697019872104E-16,3.));
#10062=CARTESIAN_POINT('Origin',(31.,0.,0.));
#10063=CARTESIAN_POINT('Origin',(0.,0.,3.));
#10064=CARTESIAN_POINT('',(1.5,-1.83697019872103E-16,5.));
#10065=CARTESIAN_POINT('Origin',(0.,0.,5.));
#10066=CARTESIAN_POINT('',(1.5,-1.83697019872103E-16,0.));
#10067=CARTESIAN_POINT('',(1.5,-1.83697019872103E-16,3.));
#10068=CARTESIAN_POINT('Origin',(0.,0.,0.));
#10069=CARTESIAN_POINT('Origin',(0.,0.,3.));
#10070=CARTESIAN_POINT('',(-3.35410196624968,1.,3.));
#10071=CARTESIAN_POINT('',(-3.35410196624968,-1.,3.));
#10072=CARTESIAN_POINT('Origin',(0.,0.,3.));
#10073=CARTESIAN_POINT('',(0.,3.5,3.));
#10074=CARTESIAN_POINT('Origin',(0.,0.,3.));
#10075=CARTESIAN_POINT('',(0.,3.5,0.));
#10076=CARTESIAN_POINT('',(0.,3.5,3.));
#10077=CARTESIAN_POINT('',(0.,-3.5,0.));
#10078=CARTESIAN_POINT('Origin',(0.,0.,0.));
#10079=CARTESIAN_POINT('',(0.,-3.5,3.));
#10080=CARTESIAN_POINT('',(0.,-3.5,3.));
#10081=CARTESIAN_POINT('Origin',(0.,0.,3.));
#10082=CARTESIAN_POINT('Origin',(0.,0.,3.));
#10083=CARTESIAN_POINT('',(-2.82842712474619,-1.,3.));
#10084=CARTESIAN_POINT('',(-2.82842712474619,1.,3.));
#10085=CARTESIAN_POINT('Origin',(0.,0.,3.));
#10086=CARTESIAN_POINT('',(0.,-1.,3.));
#10087=CARTESIAN_POINT('',(31.,-3.5,3.));
#10088=CARTESIAN_POINT('',(31.,-3.5,3.));
#10089=CARTESIAN_POINT('',(31.,3.5,3.));
#10090=CARTESIAN_POINT('Origin',(31.,0.,3.));
#10091=CARTESIAN_POINT('',(0.,3.5,3.));
#10092=CARTESIAN_POINT('',(0.,1.,3.));
#10093=CARTESIAN_POINT('',(29.197224362268,-3.,3.));
#10094=CARTESIAN_POINT('',(29.197224362268,3.,3.));
#10095=CARTESIAN_POINT('Origin',(31.,0.,3.));
#10096=CARTESIAN_POINT('',(1.802775637732,-3.,3.));
#10097=CARTESIAN_POINT('',(1.802775637732,3.,3.));
#10098=CARTESIAN_POINT('Origin',(0.,0.,0.));
#10099=CARTESIAN_POINT('',(31.,3.5,0.));
#10100=CARTESIAN_POINT('',(0.,3.5,0.));
#10101=CARTESIAN_POINT('',(31.,-3.5,0.));
#10102=CARTESIAN_POINT('Origin',(31.,0.,0.));
#10103=CARTESIAN_POINT('',(31.,-3.5,0.));
#10104=CARTESIAN_POINT('',(1.80277563773199,3.,0.));
#10105=CARTESIAN_POINT('',(1.802775637732,3.,0.));
#10106=CARTESIAN_POINT('',(1.802775637732,-3.,0.));
#10107=CARTESIAN_POINT('Origin',(0.,0.,0.));
#10108=CARTESIAN_POINT('',(1.802775637732,-3.,0.));
#10109=CARTESIAN_POINT('Origin',(31.,-3.5,3.));
#10110=CARTESIAN_POINT('',(31.,-3.5,3.));
#10111=CARTESIAN_POINT('Origin',(31.,0.,3.));
#10112=CARTESIAN_POINT('',(31.,3.5,3.));
#10113=CARTESIAN_POINT('Origin',(0.,3.5,3.));
#10114=CARTESIAN_POINT('Origin',(31.,0.,2.5));
#10115=CARTESIAN_POINT('',(29.197224362268,3.,2.5));
#10116=CARTESIAN_POINT('',(29.197224362268,3.,2.5));
#10117=CARTESIAN_POINT('',(29.197224362268,-3.,2.5));
#10118=CARTESIAN_POINT('Origin',(31.,0.,2.5));
#10119=CARTESIAN_POINT('',(29.197224362268,-3.,2.5));
#10120=CARTESIAN_POINT('Origin',(1.802775637732,-3.,2.5));
#10121=CARTESIAN_POINT('',(1.802775637732,-3.,2.5));
#10122=CARTESIAN_POINT('Origin',(1.802775637732,3.,2.5));
#10123=CARTESIAN_POINT('',(1.802775637732,3.,2.5));
#10124=CARTESIAN_POINT('Origin',(31.,0.,2.5));
#10125=CARTESIAN_POINT('Origin',(1.802775637732,3.,0.5));
#10126=CARTESIAN_POINT('',(1.80277563773199,3.,0.5));
#10127=CARTESIAN_POINT('',(1.802775637732,3.,0.5));
#10128=CARTESIAN_POINT('',(1.80277563773199,3.,0.5));
#10129=CARTESIAN_POINT('Origin',(0.,0.,0.5));
#10130=CARTESIAN_POINT('',(1.802775637732,-3.,0.5));
#10131=CARTESIAN_POINT('Origin',(0.,0.,0.5));
#10132=CARTESIAN_POINT('',(1.802775637732,-3.,0.5));
#10133=CARTESIAN_POINT('Origin',(1.802775637732,-3.,0.5));
#10134=CARTESIAN_POINT('',(1.802775637732,-3.,0.5));
#10135=CARTESIAN_POINT('Origin',(31.,0.,0.5));
#10136=CARTESIAN_POINT('Origin',(0.,0.,3.));
#10137=CARTESIAN_POINT('',(-4.,1.,3.));
#10138=CARTESIAN_POINT('',(0.,1.,3.));
#10139=CARTESIAN_POINT('',(-4.,-1.,3.));
#10140=CARTESIAN_POINT('',(0.,-1.,3.));
#10141=CARTESIAN_POINT('',(-4.,0.,3.));
#10142=CARTESIAN_POINT('Origin',(0.,-1.,5.));
#10143=CARTESIAN_POINT('',(-2.82842712474619,-1.,5.));
#10144=CARTESIAN_POINT('',(-2.82842712474619,-1.,5.));
#10145=CARTESIAN_POINT('',(-4.,-1.,5.));
#10146=CARTESIAN_POINT('',(0.,-1.,5.));
#10147=CARTESIAN_POINT('',(-4.,-1.,5.));
#10148=CARTESIAN_POINT('Origin',(0.,0.,5.));
#10149=CARTESIAN_POINT('',(-2.82842712474619,1.,5.));
#10150=CARTESIAN_POINT('',(-2.82842712474619,1.,5.));
#10151=CARTESIAN_POINT('Origin',(0.,0.,5.));
#10152=CARTESIAN_POINT('Origin',(0.,1.,5.));
#10153=CARTESIAN_POINT('',(-4.,1.,5.));
#10154=CARTESIAN_POINT('',(-4.,1.,5.));
#10155=CARTESIAN_POINT('',(0.,1.,5.));
#10156=CARTESIAN_POINT('Origin',(-4.,0.,5.));
#10157=CARTESIAN_POINT('',(-4.,0.,5.));
#10158=CARTESIAN_POINT('Origin',(0.,0.,5.));
#10159=CARTESIAN_POINT('Origin',(0.,0.,5.));
#11914=UNCERTAINTY_MEASURE_WITH_UNIT(LENGTH_MEASURE(0.01),#11934,
'DISTANCE_ACCURACY_VALUE',
'Maximum model space distance between geometric entities at asserted c
onnectivities');
#11922=UNCERTAINTY_MEASURE_WITH_UNIT(LENGTH_MEASURE(0.01),#11934,
'DISTANCE_ACCURACY_VALUE',
'Maximum model space distance between geometric entities at asserted c
onnectivities');
#11925=(
GEOMETRIC_REPRESENTATION_CONTEXT(3)
GLOBAL_UNCERTAINTY_ASSIGNED_CONTEXT((#11914))
GLOBAL_UNIT_ASSIGNED_CONTEXT((#11934,#11936,#11937))
REPRESENTATION_CONTEXT('','3D')
);
#11933=(
GEOMETRIC_REPRESENTATION_CONTEXT(3)
GLOBAL_UNCERTAINTY_ASSIGNED_CONTEXT((#11922))
GLOBAL_UNIT_ASSIGNED_CONTEXT((#11934,#11936,#11937))
REPRESENTATION_CONTEXT('','3D')
);
#11934=(
LENGTH_UNIT()
NAMED_UNIT(*)
SI_UNIT(.MILLI.,.METRE.)
);
#11936=(
NAMED_UNIT(*)
PLANE_ANGLE_UNIT()
SI_UNIT($,.RADIAN.)
);
#11937=(
NAMED_UNIT(*)
SI_UNIT($,.STERADIAN.)
SOLID_ANGLE_UNIT()
);
#11940=SHAPE_DEFINITION_REPRESENTATION(#11950,#11989);
#11950=PRODUCT_DEFINITION_SHAPE('',$,#12000);
#11989=SHAPE_REPRESENTATION('',(#6800),#11925);
#11997=PRODUCT_DEFINITION_CONTEXT('part definition',#12029,'design');
#12000=PRODUCT_DEFINITION('Short Drive Link','Short Drive Link',#12010,
#11997);
#12010=PRODUCT_DEFINITION_FORMATION('',$,#12033);
#12029=APPLICATION_CONTEXT(
'Core Data for Automotive Mechanical Design Process');
#12030=PRODUCT_CONTEXT('part definition',#12029,'mechanical');
#12033=PRODUCT('Short Drive Link','Short Drive Link',$,(#12030));
#12042=PRESENTATION_STYLE_ASSIGNMENT((#12046));
#12046=SURFACE_STYLE_USAGE(.BOTH.,#12050);
#12050=SURFACE_SIDE_STYLE('',(#12054));
#12054=SURFACE_STYLE_FILL_AREA(#12058);
#12058=FILL_AREA_STYLE('Opaque(227,224,212)',(#12062));
#12062=FILL_AREA_STYLE_COLOUR('Opaque(227,224,212)',#12066);
#12066=COLOUR_RGB('Opaque(227,224,212)',0.890196078431372,0.87843137254902,
0.831372549019608);
ENDSEC;
END-ISO-10303-21;
